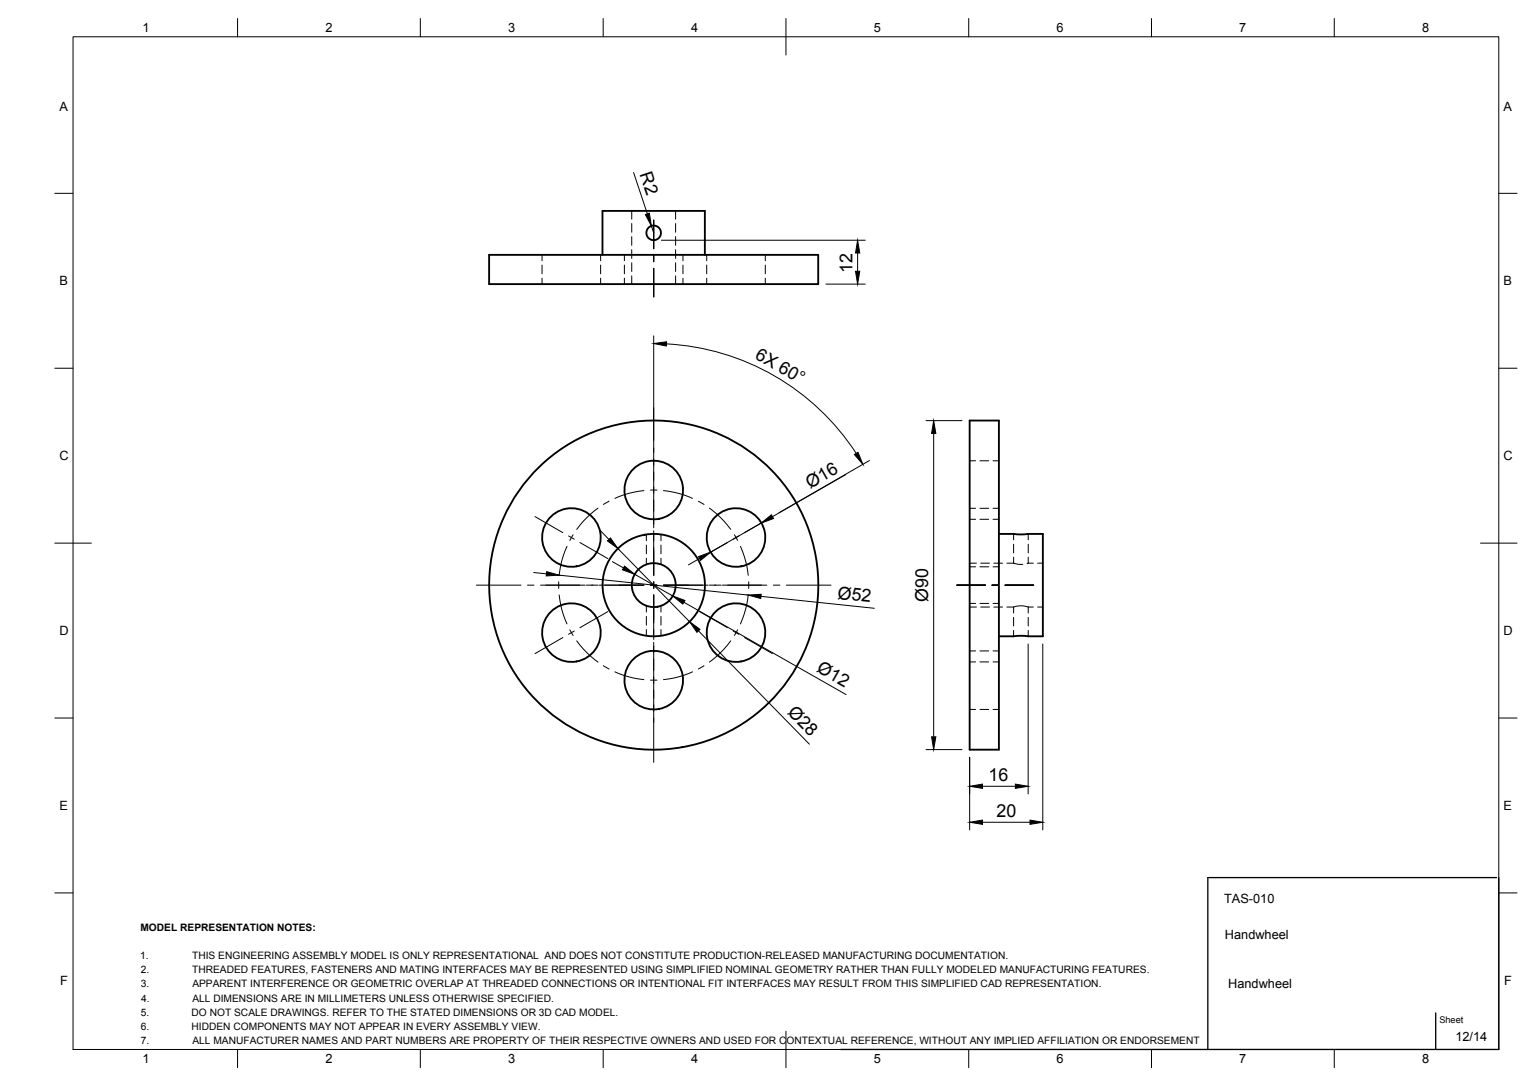
ISO-10303-21;
HEADER;
/* Generated by software containing ST-Developer
 * from STEP Tools, Inc. (www.steptools.com) 
 */

FILE_DESCRIPTION(
/* description */ (
'Independent keyed-quill tailstock, native coupled50mm slider andM16x2
 feed screw, conical dead center, bronze sleeves/thrust washers, cross
-pinned handwheel and bolted guide key. Custom center taper; no standa
rd taper compatibility, machine-bed compatibility or load rating assig
ned.'),
/* implementation_level */ '2;1');

FILE_NAME(
/* name */ 'Handwheel.step',
/* time_stamp */ '2026-11-14T07:17:36-08:00',
/* author */ (''),
/* organization */ (''),
/* preprocessor_version */ 'ST-DEVELOPER v20.2',
/* originating_system */ 'Autodesk Translation Framework v15.17.0.0',
/* authorisation */ '');

FILE_SCHEMA (('AUTOMOTIVE_DESIGN { 1 0 10303 214 3 1 1 }'));
ENDSEC;

DATA;
#10=MECHANICAL_DESIGN_GEOMETRIC_PRESENTATION_REPRESENTATION('',(#162),#289387);
#128=SHAPE_REPRESENTATION_RELATIONSHIP('SRR','None',#289463,#145);
#145=ADVANCED_BREP_SHAPE_REPRESENTATION('',(#179),#289379);
#162=STYLED_ITEM('',(#289549),#179);
#179=MANIFOLD_SOLID_BREP('Body1',#16850);
#243=FACE_BOUND('',#1657,.T.);
#244=FACE_BOUND('',#1659,.T.);
#245=FACE_BOUND('',#1661,.T.);
#246=FACE_BOUND('',#1664,.T.);
#247=FACE_BOUND('',#1665,.T.);
#248=FACE_BOUND('',#1666,.T.);
#249=FACE_BOUND('',#1667,.T.);
#250=FACE_BOUND('',#1668,.T.);
#251=FACE_BOUND('',#1669,.T.);
#252=FACE_BOUND('',#1670,.T.);
#253=FACE_BOUND('',#1672,.T.);
#254=FACE_BOUND('',#1673,.T.);
#255=FACE_BOUND('',#1674,.T.);
#256=FACE_BOUND('',#1675,.T.);
#257=FACE_BOUND('',#1676,.T.);
#258=FACE_BOUND('',#1677,.T.);
#259=FACE_BOUND('',#1678,.T.);
#377=PLANE('',#17691);
#378=PLANE('',#17698);
#379=PLANE('',#17699);
#942=FACE_OUTER_BOUND('',#1648,.T.);
#943=FACE_OUTER_BOUND('',#1649,.T.);
#944=FACE_OUTER_BOUND('',#1650,.T.);
#945=FACE_OUTER_BOUND('',#1651,.T.);
#946=FACE_OUTER_BOUND('',#1652,.T.);
#947=FACE_OUTER_BOUND('',#1653,.T.);
#948=FACE_OUTER_BOUND('',#1654,.T.);
#949=FACE_OUTER_BOUND('',#1655,.T.);
#950=FACE_OUTER_BOUND('',#1656,.T.);
#951=FACE_OUTER_BOUND('',#1658,.T.);
#952=FACE_OUTER_BOUND('',#1660,.T.);
#953=FACE_OUTER_BOUND('',#1662,.T.);
#954=FACE_OUTER_BOUND('',#1663,.T.);
#955=FACE_OUTER_BOUND('',#1671,.T.);
#1648=EDGE_LOOP('',(#14691,#14692,#14693,#14694,#14695,#14696));
#1649=EDGE_LOOP('',(#14697,#14698,#14699,#14700,#14701,#14702,#14703,#14704));
#1650=EDGE_LOOP('',(#14705,#14706,#14707,#14708));
#1651=EDGE_LOOP('',(#14709,#14710,#14711,#14712));
#1652=EDGE_LOOP('',(#14713,#14714,#14715,#14716));
#1653=EDGE_LOOP('',(#14717,#14718,#14719,#14720));
#1654=EDGE_LOOP('',(#14721,#14722,#14723,#14724));
#1655=EDGE_LOOP('',(#14725,#14726,#14727,#14728));
#1656=EDGE_LOOP('',(#14729,#14730,#14731,#14732,#14733,#14734,#14735,#14736,
#14737));
#1657=EDGE_LOOP('',(#14738,#14739,#14740));
#1658=EDGE_LOOP('',(#14741));
#1659=EDGE_LOOP('',(#14742));
#1660=EDGE_LOOP('',(#14743,#14744,#14745,#14746,#14747,#14748,#14749,#14750,
#14751));
#1661=EDGE_LOOP('',(#14752));
#1662=EDGE_LOOP('',(#14753,#14754,#14755,#14756));
#1663=EDGE_LOOP('',(#14757));
#1664=EDGE_LOOP('',(#14758));
#1665=EDGE_LOOP('',(#14759));
#1666=EDGE_LOOP('',(#14760));
#1667=EDGE_LOOP('',(#14761));
#1668=EDGE_LOOP('',(#14762));
#1669=EDGE_LOOP('',(#14763));
#1670=EDGE_LOOP('',(#14764));
#1671=EDGE_LOOP('',(#14765));
#1672=EDGE_LOOP('',(#14766));
#1673=EDGE_LOOP('',(#14767));
#1674=EDGE_LOOP('',(#14768));
#1675=EDGE_LOOP('',(#14769));
#1676=EDGE_LOOP('',(#14770));
#1677=EDGE_LOOP('',(#14771));
#1678=EDGE_LOOP('',(#14772));
#1925=CIRCLE('',#17671,8.);
#1926=CIRCLE('',#17672,8.);
#1927=CIRCLE('',#17674,8.);
#1928=CIRCLE('',#17675,8.);
#1929=CIRCLE('',#17677,8.);
#1930=CIRCLE('',#17678,8.);
#1931=CIRCLE('',#17680,8.);
#1932=CIRCLE('',#17681,8.);
#1933=CIRCLE('',#17683,8.);
#1934=CIRCLE('',#17684,8.);
#1935=CIRCLE('',#17686,8.);
#1936=CIRCLE('',#17687,8.);
#1937=CIRCLE('',#17689,14.);
#1938=CIRCLE('',#17690,14.);
#1939=CIRCLE('',#17692,6.);
#1940=CIRCLE('',#17694,6.);
#1941=CIRCLE('',#17696,45.);
#1942=CIRCLE('',#17697,45.);
#3636=B_SPLINE_CURVE_WITH_KNOTS('',3,(#247043,#247044,#247045,#247046,#247047,
#247048,#247049,#247050,#247051,#247052),.UNSPECIFIED.,.F.,.F.,(4,2,2,2,
4),(0.905379612473188,0.980827373439309,1.05627513440543,1.13172397551817,
1.20717281663092),.UNSPECIFIED.);
#3637=B_SPLINE_CURVE_WITH_KNOTS('',3,(#247054,#247055,#247056,#247057,#247058,
#247059,#247060,#247061,#247062,#247063,#247064,#247065,#247066,#247067,
#247068,#247069,#247070,#247071),.UNSPECIFIED.,.F.,.F.,(4,2,2,2,2,2,2,2,
4),(0.301793204157729,0.377240965123851,0.452688726089972,0.528137567202715,
0.603586408315459,0.679035249428202,0.754484090540945,0.829931851507066,
0.905379612473188),.UNSPECIFIED.);
#3638=B_SPLINE_CURVE_WITH_KNOTS('',3,(#247072,#247073,#247074,#247075,#247076,
#247077,#247078,#247079,#247080,#247081),.UNSPECIFIED.,.F.,.F.,(4,2,2,2,
4),(1.20717281663092,1.28262165774366,1.3580704988564,1.43351825982252,
1.50896602078865),.UNSPECIFIED.);
#3639=B_SPLINE_CURVE_WITH_KNOTS('',3,(#247084,#247085,#247086,#247087,#247088,
#247089,#247090,#247091,#247092,#247093,#247094,#247095,#247096,#247097,
#247098,#247099,#247100,#247101,#247102,#247103,#247104,#247105,#247106,
#247107,#247108,#247109,#247110,#247111,#247112,#247113,#247114,#247115,
#247116,#247117),.UNSPECIFIED.,.T.,.F.,(4,2,2,2,2,2,2,2,2,2,2,2,2,2,2,2,
4),(-1.21552023492118,-1.13953259867645,-1.06354496243171,-0.987592569311299,
-0.911640176190888,-0.835687783070478,-0.759735389950067,-0.683747753705329,
-0.607760117460592,-0.531772481215855,-0.455784844971118,-0.379832451850707,
-0.303880058730296,-0.227927665609885,-0.151975272489474,-0.0759876362447371,
0.),.UNSPECIFIED.);
#3640=B_SPLINE_CURVE_WITH_KNOTS('',3,(#247121,#247122,#247123,#247124,#247125,
#247126,#247127,#247128,#247129,#247130),.UNSPECIFIED.,.F.,.F.,(4,2,2,2,
4),(-0.303880058730296,-0.227927665609886,-0.151975272489475,-0.0759876362447375,
0.),.UNSPECIFIED.);
#3641=B_SPLINE_CURVE_WITH_KNOTS('',3,(#247132,#247133,#247134,#247135,#247136,
#247137,#247138,#247139,#247140,#247141,#247142,#247143,#247144,#247145,
#247146,#247147,#247148,#247149),.UNSPECIFIED.,.F.,.F.,(4,2,2,2,2,2,2,2,
4),(-0.911640176190889,-0.835687783070478,-0.759735389950067,-0.68374775370533,
-0.607760117460593,-0.531772481215855,-0.455784844971118,-0.379832451850707,
-0.303880058730296),.UNSPECIFIED.);
#3642=B_SPLINE_CURVE_WITH_KNOTS('',3,(#247150,#247151,#247152,#247153,#247154,
#247155,#247156,#247157,#247158,#247159),.UNSPECIFIED.,.F.,.F.,(4,2,2,2,
4),(0.,0.0759876362447371,0.151975272489474,0.227927665609885,0.303880058730296),
 .UNSPECIFIED.);
#3643=B_SPLINE_CURVE_WITH_KNOTS('',3,(#247163,#247164,#247165,#247166,#247167,
#247168,#247169,#247170,#247171,#247172),.UNSPECIFIED.,.F.,.F.,(4,2,2,2,
4),(0.905379612473188,0.980827373439309,1.05627513440543,1.13172397551817,
1.20717281663092),.UNSPECIFIED.);
#3644=B_SPLINE_CURVE_WITH_KNOTS('',3,(#247174,#247175,#247176,#247177,#247178,
#247179,#247180,#247181,#247182,#247183,#247184,#247185,#247186,#247187,
#247188,#247189,#247190,#247191),.UNSPECIFIED.,.F.,.F.,(4,2,2,2,2,2,2,2,
4),(0.301793204157729,0.377240965123851,0.452688726089972,0.528137567202715,
0.603586408315459,0.679035249428202,0.754484090540945,0.829931851507066,
0.905379612473188),.UNSPECIFIED.);
#3645=B_SPLINE_CURVE_WITH_KNOTS('',3,(#247192,#247193,#247194,#247195,#247196,
#247197,#247198,#247199,#247200,#247201),.UNSPECIFIED.,.F.,.F.,(4,2,2,2,
4),(1.20717281663092,1.28262165774366,1.3580704988564,1.43351825982252,
1.50896602078865),.UNSPECIFIED.);
#4443=LINE('',#247083,#5080);
#4444=LINE('',#247161,#5081);
#4445=LINE('',#247206,#5082);
#4446=LINE('',#247212,#5083);
#4447=LINE('',#247218,#5084);
#4448=LINE('',#247224,#5085);
#4449=LINE('',#247230,#5086);
#4450=LINE('',#247236,#5087);
#4451=LINE('',#247241,#5088);
#4452=LINE('',#247243,#5089);
#4453=LINE('',#247251,#5090);
#4454=LINE('',#247252,#5091);
#4455=LINE('',#247257,#5092);
#5080=VECTOR('',#19637,2.);
#5081=VECTOR('',#19640,2.);
#5082=VECTOR('',#19645,8.);
#5083=VECTOR('',#19652,8.);
#5084=VECTOR('',#19659,8.);
#5085=VECTOR('',#19666,8.);
#5086=VECTOR('',#19673,8.);
#5087=VECTOR('',#19680,8.);
#5088=VECTOR('',#19687,14.);
#5089=VECTOR('',#19688,14.);
#5090=VECTOR('',#19699,6.);
#5091=VECTOR('',#19700,6.);
#5092=VECTOR('',#19705,45.);
#6995=VERTEX_POINT('',#247041);
#6996=VERTEX_POINT('',#247042);
#6997=VERTEX_POINT('',#247053);
#6998=VERTEX_POINT('',#247082);
#6999=VERTEX_POINT('',#247119);
#7000=VERTEX_POINT('',#247120);
#7001=VERTEX_POINT('',#247131);
#7002=VERTEX_POINT('',#247160);
#7003=VERTEX_POINT('',#247162);
#7004=VERTEX_POINT('',#247173);
#7005=VERTEX_POINT('',#247203);
#7006=VERTEX_POINT('',#247205);
#7007=VERTEX_POINT('',#247209);
#7008=VERTEX_POINT('',#247211);
#7009=VERTEX_POINT('',#247215);
#7010=VERTEX_POINT('',#247217);
#7011=VERTEX_POINT('',#247221);
#7012=VERTEX_POINT('',#247223);
#7013=VERTEX_POINT('',#247227);
#7014=VERTEX_POINT('',#247229);
#7015=VERTEX_POINT('',#247233);
#7016=VERTEX_POINT('',#247235);
#7017=VERTEX_POINT('',#247239);
#7018=VERTEX_POINT('',#247242);
#7019=VERTEX_POINT('',#247246);
#7020=VERTEX_POINT('',#247249);
#7021=VERTEX_POINT('',#247254);
#7022=VERTEX_POINT('',#247256);
#9657=EDGE_CURVE('',#6995,#6996,#3636,.T.);
#9658=EDGE_CURVE('',#6997,#6995,#3637,.T.);
#9659=EDGE_CURVE('',#6996,#6997,#3638,.T.);
#9660=EDGE_CURVE('',#6996,#6998,#4443,.T.);
#9661=EDGE_CURVE('',#6998,#6998,#3639,.T.);
#9662=EDGE_CURVE('',#6999,#7000,#3640,.T.);
#9663=EDGE_CURVE('',#7001,#6999,#3641,.T.);
#9664=EDGE_CURVE('',#7000,#7001,#3642,.T.);
#9665=EDGE_CURVE('',#7000,#7002,#4444,.T.);
#9666=EDGE_CURVE('',#7003,#7002,#3643,.T.);
#9667=EDGE_CURVE('',#7004,#7003,#3644,.T.);
#9668=EDGE_CURVE('',#7002,#7004,#3645,.T.);
#9669=EDGE_CURVE('',#7005,#7005,#1925,.T.);
#9670=EDGE_CURVE('',#7005,#7006,#4445,.T.);
#9671=EDGE_CURVE('',#7006,#7006,#1926,.T.);
#9672=EDGE_CURVE('',#7007,#7007,#1927,.T.);
#9673=EDGE_CURVE('',#7007,#7008,#4446,.T.);
#9674=EDGE_CURVE('',#7008,#7008,#1928,.T.);
#9675=EDGE_CURVE('',#7009,#7009,#1929,.T.);
#9676=EDGE_CURVE('',#7009,#7010,#4447,.T.);
#9677=EDGE_CURVE('',#7010,#7010,#1930,.T.);
#9678=EDGE_CURVE('',#7011,#7011,#1931,.T.);
#9679=EDGE_CURVE('',#7011,#7012,#4448,.T.);
#9680=EDGE_CURVE('',#7012,#7012,#1932,.T.);
#9681=EDGE_CURVE('',#7013,#7013,#1933,.T.);
#9682=EDGE_CURVE('',#7013,#7014,#4449,.T.);
#9683=EDGE_CURVE('',#7014,#7014,#1934,.T.);
#9684=EDGE_CURVE('',#7015,#7015,#1935,.T.);
#9685=EDGE_CURVE('',#7015,#7016,#4450,.T.);
#9686=EDGE_CURVE('',#7016,#7016,#1936,.T.);
#9687=EDGE_CURVE('',#7017,#7017,#1937,.T.);
#9688=EDGE_CURVE('',#7017,#7003,#4451,.T.);
#9689=EDGE_CURVE('',#7004,#7018,#4452,.T.);
#9690=EDGE_CURVE('',#7018,#7018,#1938,.T.);
#9691=EDGE_CURVE('',#7019,#7019,#1939,.T.);
#9692=EDGE_CURVE('',#7020,#7020,#1940,.T.);
#9693=EDGE_CURVE('',#7020,#6999,#4453,.T.);
#9694=EDGE_CURVE('',#7001,#7019,#4454,.T.);
#9695=EDGE_CURVE('',#7021,#7021,#1941,.F.);
#9696=EDGE_CURVE('',#7021,#7022,#4455,.T.);
#9697=EDGE_CURVE('',#7022,#7022,#1942,.F.);
#14691=ORIENTED_EDGE('',*,*,#9657,.F.);
#14692=ORIENTED_EDGE('',*,*,#9658,.F.);
#14693=ORIENTED_EDGE('',*,*,#9659,.F.);
#14694=ORIENTED_EDGE('',*,*,#9660,.T.);
#14695=ORIENTED_EDGE('',*,*,#9661,.F.);
#14696=ORIENTED_EDGE('',*,*,#9660,.F.);
#14697=ORIENTED_EDGE('',*,*,#9662,.F.);
#14698=ORIENTED_EDGE('',*,*,#9663,.F.);
#14699=ORIENTED_EDGE('',*,*,#9664,.F.);
#14700=ORIENTED_EDGE('',*,*,#9665,.T.);
#14701=ORIENTED_EDGE('',*,*,#9666,.F.);
#14702=ORIENTED_EDGE('',*,*,#9667,.F.);
#14703=ORIENTED_EDGE('',*,*,#9668,.F.);
#14704=ORIENTED_EDGE('',*,*,#9665,.F.);
#14705=ORIENTED_EDGE('',*,*,#9669,.F.);
#14706=ORIENTED_EDGE('',*,*,#9670,.T.);
#14707=ORIENTED_EDGE('',*,*,#9671,.F.);
#14708=ORIENTED_EDGE('',*,*,#9670,.F.);
#14709=ORIENTED_EDGE('',*,*,#9672,.F.);
#14710=ORIENTED_EDGE('',*,*,#9673,.T.);
#14711=ORIENTED_EDGE('',*,*,#9674,.F.);
#14712=ORIENTED_EDGE('',*,*,#9673,.F.);
#14713=ORIENTED_EDGE('',*,*,#9675,.F.);
#14714=ORIENTED_EDGE('',*,*,#9676,.T.);
#14715=ORIENTED_EDGE('',*,*,#9677,.F.);
#14716=ORIENTED_EDGE('',*,*,#9676,.F.);
#14717=ORIENTED_EDGE('',*,*,#9678,.F.);
#14718=ORIENTED_EDGE('',*,*,#9679,.T.);
#14719=ORIENTED_EDGE('',*,*,#9680,.F.);
#14720=ORIENTED_EDGE('',*,*,#9679,.F.);
#14721=ORIENTED_EDGE('',*,*,#9681,.F.);
#14722=ORIENTED_EDGE('',*,*,#9682,.T.);
#14723=ORIENTED_EDGE('',*,*,#9683,.F.);
#14724=ORIENTED_EDGE('',*,*,#9682,.F.);
#14725=ORIENTED_EDGE('',*,*,#9684,.F.);
#14726=ORIENTED_EDGE('',*,*,#9685,.T.);
#14727=ORIENTED_EDGE('',*,*,#9686,.F.);
#14728=ORIENTED_EDGE('',*,*,#9685,.F.);
#14729=ORIENTED_EDGE('',*,*,#9687,.F.);
#14730=ORIENTED_EDGE('',*,*,#9688,.T.);
#14731=ORIENTED_EDGE('',*,*,#9666,.T.);
#14732=ORIENTED_EDGE('',*,*,#9668,.T.);
#14733=ORIENTED_EDGE('',*,*,#9689,.T.);
#14734=ORIENTED_EDGE('',*,*,#9690,.F.);
#14735=ORIENTED_EDGE('',*,*,#9689,.F.);
#14736=ORIENTED_EDGE('',*,*,#9667,.T.);
#14737=ORIENTED_EDGE('',*,*,#9688,.F.);
#14738=ORIENTED_EDGE('',*,*,#9658,.T.);
#14739=ORIENTED_EDGE('',*,*,#9657,.T.);
#14740=ORIENTED_EDGE('',*,*,#9659,.T.);
#14741=ORIENTED_EDGE('',*,*,#9687,.T.);
#14742=ORIENTED_EDGE('',*,*,#9691,.T.);
#14743=ORIENTED_EDGE('',*,*,#9692,.T.);
#14744=ORIENTED_EDGE('',*,*,#9693,.T.);
#14745=ORIENTED_EDGE('',*,*,#9662,.T.);
#14746=ORIENTED_EDGE('',*,*,#9664,.T.);
#14747=ORIENTED_EDGE('',*,*,#9694,.T.);
#14748=ORIENTED_EDGE('',*,*,#9691,.F.);
#14749=ORIENTED_EDGE('',*,*,#9694,.F.);
#14750=ORIENTED_EDGE('',*,*,#9663,.T.);
#14751=ORIENTED_EDGE('',*,*,#9693,.F.);
#14752=ORIENTED_EDGE('',*,*,#9661,.T.);
#14753=ORIENTED_EDGE('',*,*,#9695,.F.);
#14754=ORIENTED_EDGE('',*,*,#9696,.T.);
#14755=ORIENTED_EDGE('',*,*,#9697,.T.);
#14756=ORIENTED_EDGE('',*,*,#9696,.F.);
#14757=ORIENTED_EDGE('',*,*,#9695,.T.);
#14758=ORIENTED_EDGE('',*,*,#9690,.T.);
#14759=ORIENTED_EDGE('',*,*,#9684,.T.);
#14760=ORIENTED_EDGE('',*,*,#9681,.T.);
#14761=ORIENTED_EDGE('',*,*,#9678,.T.);
#14762=ORIENTED_EDGE('',*,*,#9675,.T.);
#14763=ORIENTED_EDGE('',*,*,#9672,.T.);
#14764=ORIENTED_EDGE('',*,*,#9669,.T.);
#14765=ORIENTED_EDGE('',*,*,#9697,.F.);
#14766=ORIENTED_EDGE('',*,*,#9692,.F.);
#14767=ORIENTED_EDGE('',*,*,#9686,.T.);
#14768=ORIENTED_EDGE('',*,*,#9683,.T.);
#14769=ORIENTED_EDGE('',*,*,#9680,.T.);
#14770=ORIENTED_EDGE('',*,*,#9677,.T.);
#14771=ORIENTED_EDGE('',*,*,#9674,.T.);
#14772=ORIENTED_EDGE('',*,*,#9671,.T.);
#16117=CYLINDRICAL_SURFACE('',#17668,2.);
#16118=CYLINDRICAL_SURFACE('',#17669,2.);
#16119=CYLINDRICAL_SURFACE('',#17670,8.);
#16120=CYLINDRICAL_SURFACE('',#17673,8.);
#16121=CYLINDRICAL_SURFACE('',#17676,8.);
#16122=CYLINDRICAL_SURFACE('',#17679,8.);
#16123=CYLINDRICAL_SURFACE('',#17682,8.);
#16124=CYLINDRICAL_SURFACE('',#17685,8.);
#16125=CYLINDRICAL_SURFACE('',#17688,14.);
#16126=CYLINDRICAL_SURFACE('',#17693,6.);
#16127=CYLINDRICAL_SURFACE('',#17695,45.);
#16710=ADVANCED_FACE('',(#942),#16117,.F.);
#16711=ADVANCED_FACE('',(#943),#16118,.F.);
#16712=ADVANCED_FACE('',(#944),#16119,.F.);
#16713=ADVANCED_FACE('',(#945),#16120,.F.);
#16714=ADVANCED_FACE('',(#946),#16121,.F.);
#16715=ADVANCED_FACE('',(#947),#16122,.F.);
#16716=ADVANCED_FACE('',(#948),#16123,.F.);
#16717=ADVANCED_FACE('',(#949),#16124,.F.);
#16718=ADVANCED_FACE('',(#950,#243),#16125,.T.);
#16719=ADVANCED_FACE('',(#951,#244),#377,.T.);
#16720=ADVANCED_FACE('',(#952,#245),#16126,.F.);
#16721=ADVANCED_FACE('',(#953),#16127,.T.);
#16722=ADVANCED_FACE('',(#954,#246,#247,#248,#249,#250,#251,#252),#378,
 .T.);
#16723=ADVANCED_FACE('',(#955,#253,#254,#255,#256,#257,#258,#259),#379,
 .F.);
#16850=CLOSED_SHELL('',(#16710,#16711,#16712,#16713,#16714,#16715,#16716,
#16717,#16718,#16719,#16720,#16721,#16722,#16723));
#17667=AXIS2_PLACEMENT_3D('',#247039,#19633,#19634);
#17668=AXIS2_PLACEMENT_3D('',#247040,#19635,#19636);
#17669=AXIS2_PLACEMENT_3D('',#247118,#19638,#19639);
#17670=AXIS2_PLACEMENT_3D('',#247202,#19641,#19642);
#17671=AXIS2_PLACEMENT_3D('',#247204,#19643,#19644);
#17672=AXIS2_PLACEMENT_3D('',#247207,#19646,#19647);
#17673=AXIS2_PLACEMENT_3D('',#247208,#19648,#19649);
#17674=AXIS2_PLACEMENT_3D('',#247210,#19650,#19651);
#17675=AXIS2_PLACEMENT_3D('',#247213,#19653,#19654);
#17676=AXIS2_PLACEMENT_3D('',#247214,#19655,#19656);
#17677=AXIS2_PLACEMENT_3D('',#247216,#19657,#19658);
#17678=AXIS2_PLACEMENT_3D('',#247219,#19660,#19661);
#17679=AXIS2_PLACEMENT_3D('',#247220,#19662,#19663);
#17680=AXIS2_PLACEMENT_3D('',#247222,#19664,#19665);
#17681=AXIS2_PLACEMENT_3D('',#247225,#19667,#19668);
#17682=AXIS2_PLACEMENT_3D('',#247226,#19669,#19670);
#17683=AXIS2_PLACEMENT_3D('',#247228,#19671,#19672);
#17684=AXIS2_PLACEMENT_3D('',#247231,#19674,#19675);
#17685=AXIS2_PLACEMENT_3D('',#247232,#19676,#19677);
#17686=AXIS2_PLACEMENT_3D('',#247234,#19678,#19679);
#17687=AXIS2_PLACEMENT_3D('',#247237,#19681,#19682);
#17688=AXIS2_PLACEMENT_3D('',#247238,#19683,#19684);
#17689=AXIS2_PLACEMENT_3D('',#247240,#19685,#19686);
#17690=AXIS2_PLACEMENT_3D('',#247244,#19689,#19690);
#17691=AXIS2_PLACEMENT_3D('',#247245,#19691,#19692);
#17692=AXIS2_PLACEMENT_3D('',#247247,#19693,#19694);
#17693=AXIS2_PLACEMENT_3D('',#247248,#19695,#19696);
#17694=AXIS2_PLACEMENT_3D('',#247250,#19697,#19698);
#17695=AXIS2_PLACEMENT_3D('',#247253,#19701,#19702);
#17696=AXIS2_PLACEMENT_3D('',#247255,#19703,#19704);
#17697=AXIS2_PLACEMENT_3D('',#247258,#19706,#19707);
#17698=AXIS2_PLACEMENT_3D('',#247259,#19708,#19709);
#17699=AXIS2_PLACEMENT_3D('',#247260,#19710,#19711);
#19633=DIRECTION('axis',(0.,0.,1.));
#19634=DIRECTION('refdir',(1.,0.,0.));
#19635=DIRECTION('center_axis',(-1.,0.,0.));
#19636=DIRECTION('ref_axis',(0.,1.,0.));
#19637=DIRECTION('',(-1.,0.,0.));
#19638=DIRECTION('center_axis',(-1.,0.,0.));
#19639=DIRECTION('ref_axis',(0.,1.,0.));
#19640=DIRECTION('',(-1.,0.,0.));
#19641=DIRECTION('center_axis',(0.,0.,-1.));
#19642=DIRECTION('ref_axis',(1.,0.,0.));
#19643=DIRECTION('center_axis',(0.,0.,-1.));
#19644=DIRECTION('ref_axis',(1.,0.,0.));
#19645=DIRECTION('',(0.,0.,-1.));
#19646=DIRECTION('center_axis',(0.,0.,1.));
#19647=DIRECTION('ref_axis',(1.,0.,0.));
#19648=DIRECTION('center_axis',(0.,0.,-1.));
#19649=DIRECTION('ref_axis',(1.,0.,0.));
#19650=DIRECTION('center_axis',(0.,0.,-1.));
#19651=DIRECTION('ref_axis',(1.,0.,0.));
#19652=DIRECTION('',(0.,0.,-1.));
#19653=DIRECTION('center_axis',(0.,0.,1.));
#19654=DIRECTION('ref_axis',(1.,0.,0.));
#19655=DIRECTION('center_axis',(0.,0.,-1.));
#19656=DIRECTION('ref_axis',(1.,0.,0.));
#19657=DIRECTION('center_axis',(0.,0.,-1.));
#19658=DIRECTION('ref_axis',(1.,0.,0.));
#19659=DIRECTION('',(0.,0.,-1.));
#19660=DIRECTION('center_axis',(0.,0.,1.));
#19661=DIRECTION('ref_axis',(1.,0.,0.));
#19662=DIRECTION('center_axis',(0.,0.,-1.));
#19663=DIRECTION('ref_axis',(1.,0.,0.));
#19664=DIRECTION('center_axis',(0.,0.,-1.));
#19665=DIRECTION('ref_axis',(1.,0.,0.));
#19666=DIRECTION('',(0.,0.,-1.));
#19667=DIRECTION('center_axis',(0.,0.,1.));
#19668=DIRECTION('ref_axis',(1.,0.,0.));
#19669=DIRECTION('center_axis',(0.,0.,-1.));
#19670=DIRECTION('ref_axis',(1.,0.,0.));
#19671=DIRECTION('center_axis',(0.,0.,-1.));
#19672=DIRECTION('ref_axis',(1.,0.,0.));
#19673=DIRECTION('',(0.,0.,-1.));
#19674=DIRECTION('center_axis',(0.,0.,1.));
#19675=DIRECTION('ref_axis',(1.,0.,0.));
#19676=DIRECTION('center_axis',(0.,0.,-1.));
#19677=DIRECTION('ref_axis',(1.,0.,0.));
#19678=DIRECTION('center_axis',(0.,0.,-1.));
#19679=DIRECTION('ref_axis',(1.,0.,0.));
#19680=DIRECTION('',(0.,0.,-1.));
#19681=DIRECTION('center_axis',(0.,0.,1.));
#19682=DIRECTION('ref_axis',(1.,0.,0.));
#19683=DIRECTION('center_axis',(0.,0.,1.));
#19684=DIRECTION('ref_axis',(1.,0.,0.));
#19685=DIRECTION('center_axis',(0.,0.,1.));
#19686=DIRECTION('ref_axis',(1.,0.,0.));
#19687=DIRECTION('',(0.,0.,-1.));
#19688=DIRECTION('',(0.,0.,-1.));
#19689=DIRECTION('center_axis',(0.,0.,-1.));
#19690=DIRECTION('ref_axis',(1.,0.,0.));
#19691=DIRECTION('center_axis',(0.,0.,1.));
#19692=DIRECTION('ref_axis',(1.,0.,0.));
#19693=DIRECTION('center_axis',(0.,0.,-1.));
#19694=DIRECTION('ref_axis',(1.,0.,0.));
#19695=DIRECTION('center_axis',(0.,0.,1.));
#19696=DIRECTION('ref_axis',(1.,0.,0.));
#19697=DIRECTION('center_axis',(0.,0.,-1.));
#19698=DIRECTION('ref_axis',(1.,0.,0.));
#19699=DIRECTION('',(0.,0.,1.));
#19700=DIRECTION('',(0.,0.,1.));
#19701=DIRECTION('center_axis',(0.,0.,1.));
#19702=DIRECTION('ref_axis',(1.,0.,0.));
#19703=DIRECTION('center_axis',(0.,0.,-1.));
#19704=DIRECTION('ref_axis',(1.,0.,0.));
#19705=DIRECTION('',(0.,0.,-1.));
#19706=DIRECTION('center_axis',(0.,0.,-1.));
#19707=DIRECTION('ref_axis',(1.,0.,0.));
#19708=DIRECTION('center_axis',(0.,0.,1.));
#19709=DIRECTION('ref_axis',(1.,0.,0.));
#19710=DIRECTION('center_axis',(0.,0.,1.));
#19711=DIRECTION('ref_axis',(1.,0.,0.));
#247039=CARTESIAN_POINT('',(0.,0.,0.));
#247040=CARTESIAN_POINT('Origin',(-2.22044604925031E-15,0.,14.));
#247041=CARTESIAN_POINT('',(14.,0.,12.));
#247042=CARTESIAN_POINT('',(13.856406460551,-2.,14.));
#247043=CARTESIAN_POINT('Ctrl Pts',(14.,6.24500451351651E-16,12.));
#247044=CARTESIAN_POINT('Ctrl Pts',(14.,-0.251492536553737,12.));
#247045=CARTESIAN_POINT('Ctrl Pts',(13.992532457489,-0.519514815600169,
12.0503312082537));
#247046=CARTESIAN_POINT('Ctrl Pts',(13.965542073511,-1.01217331161422,12.2545461305954));
#247047=CARTESIAN_POINT('Ctrl Pts',(13.9463980317977,-1.23683805013847,
12.4084109253923));
#247048=CARTESIAN_POINT('Ctrl Pts',(13.9103782647342,-1.59159161400131,
12.7631644892551));
#247049=CARTESIAN_POINT('Ctrl Pts',(13.891148239315,-1.74545441720186,12.9878281297258));
#247050=CARTESIAN_POINT('Ctrl Pts',(13.8639606805058,-1.94966788779478,
13.4804828838555));
#247051=CARTESIAN_POINT('Ctrl Pts',(13.856406460551,-2.,13.7485038629575));
#247052=CARTESIAN_POINT('Ctrl Pts',(13.856406460551,-2.,14.));
#247053=CARTESIAN_POINT('',(14.,0.,16.));
#247054=CARTESIAN_POINT('Ctrl Pts',(14.,-2.77555756156289E-16,16.));
#247055=CARTESIAN_POINT('Ctrl Pts',(14.,0.251492536553738,16.));
#247056=CARTESIAN_POINT('Ctrl Pts',(13.992532457489,0.51951481560017,15.9496687917463));
#247057=CARTESIAN_POINT('Ctrl Pts',(13.965542073511,1.01217331161422,15.7454538694046));
#247058=CARTESIAN_POINT('Ctrl Pts',(13.9463980317977,1.23683805013847,15.5915890746077));
#247059=CARTESIAN_POINT('Ctrl Pts',(13.9103782647342,1.59159161400131,15.2368355107449));
#247060=CARTESIAN_POINT('Ctrl Pts',(13.891148239315,1.74545441720186,15.0121718702742));
#247061=CARTESIAN_POINT('Ctrl Pts',(13.8639606805058,1.94966788779478,14.5195171161445));
#247062=CARTESIAN_POINT('Ctrl Pts',(13.856406460551,2.,14.2514961370425));
#247063=CARTESIAN_POINT('Ctrl Pts',(13.856406460551,2.,13.7485038629575));
#247064=CARTESIAN_POINT('Ctrl Pts',(13.8639606805058,1.94966788779478,13.4804828838555));
#247065=CARTESIAN_POINT('Ctrl Pts',(13.891148239315,1.74545441720186,12.9878281297258));
#247066=CARTESIAN_POINT('Ctrl Pts',(13.9103782647342,1.59159161400131,12.7631644892551));
#247067=CARTESIAN_POINT('Ctrl Pts',(13.9463980317977,1.23683805013847,12.4084109253923));
#247068=CARTESIAN_POINT('Ctrl Pts',(13.965542073511,1.01217331161422,12.2545461305954));
#247069=CARTESIAN_POINT('Ctrl Pts',(13.992532457489,0.519514815600173,12.0503312082537));
#247070=CARTESIAN_POINT('Ctrl Pts',(14.,0.251492536553739,12.));
#247071=CARTESIAN_POINT('Ctrl Pts',(14.,6.41847686111419E-16,12.));
#247072=CARTESIAN_POINT('Ctrl Pts',(13.856406460551,-2.,14.));
#247073=CARTESIAN_POINT('Ctrl Pts',(13.856406460551,-2.,14.2514961370425));
#247074=CARTESIAN_POINT('Ctrl Pts',(13.8639606805058,-1.94966788779478,
14.5195171161445));
#247075=CARTESIAN_POINT('Ctrl Pts',(13.891148239315,-1.74545441720186,15.0121718702742));
#247076=CARTESIAN_POINT('Ctrl Pts',(13.9103782647342,-1.59159161400131,
15.2368355107449));
#247077=CARTESIAN_POINT('Ctrl Pts',(13.9463980317977,-1.23683805013847,
15.5915890746077));
#247078=CARTESIAN_POINT('Ctrl Pts',(13.965542073511,-1.01217331161422,15.7454538694046));
#247079=CARTESIAN_POINT('Ctrl Pts',(13.992532457489,-0.519514815600171,
15.9496687917463));
#247080=CARTESIAN_POINT('Ctrl Pts',(14.,-0.251492536553739,16.));
#247081=CARTESIAN_POINT('Ctrl Pts',(14.,5.03069808033274E-16,16.));
#247082=CARTESIAN_POINT('',(5.65685424949238,-2.,14.));
#247083=CARTESIAN_POINT('',(-2.22044604925031E-15,-2.,14.));
#247084=CARTESIAN_POINT('Ctrl Pts',(5.65685424949238,-2.,14.));
#247085=CARTESIAN_POINT('Ctrl Pts',(5.65685424949238,-2.,13.7467078791842));
#247086=CARTESIAN_POINT('Ctrl Pts',(5.67565356574251,-1.94898067853762,
13.477996053073));
#247087=CARTESIAN_POINT('Ctrl Pts',(5.74186082552466,-1.7443058152527,12.9858936400846));
#247088=CARTESIAN_POINT('Ctrl Pts',(5.78813771212597,-1.59074095999941,
12.7623138352532));
#247089=CARTESIAN_POINT('Ctrl Pts',(5.87374622031365,-1.23776803829002,
12.4093409135438));
#247090=CARTESIAN_POINT('Ctrl Pts',(5.9188739106068,-1.01415562391481,12.2557130277668));
#247091=CARTESIAN_POINT('Ctrl Pts',(5.98240475886912,-0.521932274441715,
12.0509911583939));
#247092=CARTESIAN_POINT('Ctrl Pts',(6.,-0.253174643734702,12.));
#247093=CARTESIAN_POINT('Ctrl Pts',(6.,0.253174643734703,12.));
#247094=CARTESIAN_POINT('Ctrl Pts',(5.98240475886912,0.521932274441715,
12.0509911583939));
#247095=CARTESIAN_POINT('Ctrl Pts',(5.9188739106068,1.01415562391481,12.2557130277668));
#247096=CARTESIAN_POINT('Ctrl Pts',(5.87374622031365,1.23776803829002,12.4093409135438));
#247097=CARTESIAN_POINT('Ctrl Pts',(5.78813771212597,1.59074095999941,12.7623138352532));
#247098=CARTESIAN_POINT('Ctrl Pts',(5.74186082552466,1.7443058152527,12.9858936400846));
#247099=CARTESIAN_POINT('Ctrl Pts',(5.67565356574251,1.94898067853762,13.477996053073));
#247100=CARTESIAN_POINT('Ctrl Pts',(5.65685424949238,2.,13.7467078791842));
#247101=CARTESIAN_POINT('Ctrl Pts',(5.65685424949238,2.,14.2532921208158));
#247102=CARTESIAN_POINT('Ctrl Pts',(5.67565356574251,1.94898067853763,14.522003946927));
#247103=CARTESIAN_POINT('Ctrl Pts',(5.74186082552466,1.74430581525271,15.0141063599154));
#247104=CARTESIAN_POINT('Ctrl Pts',(5.78813771212597,1.59074095999941,15.2376861647468));
#247105=CARTESIAN_POINT('Ctrl Pts',(5.87374622031365,1.23776803829002,15.5906590864562));
#247106=CARTESIAN_POINT('Ctrl Pts',(5.9188739106068,1.01415562391481,15.7442869722332));
#247107=CARTESIAN_POINT('Ctrl Pts',(5.98240475886912,0.521932274441714,
15.9490088416061));
#247108=CARTESIAN_POINT('Ctrl Pts',(6.,0.253174643734703,16.));
#247109=CARTESIAN_POINT('Ctrl Pts',(6.,-0.253174643734703,16.));
#247110=CARTESIAN_POINT('Ctrl Pts',(5.98240475886912,-0.521932274441715,
15.9490088416061));
#247111=CARTESIAN_POINT('Ctrl Pts',(5.9188739106068,-1.01415562391481,15.7442869722332));
#247112=CARTESIAN_POINT('Ctrl Pts',(5.87374622031365,-1.23776803829002,
15.5906590864562));
#247113=CARTESIAN_POINT('Ctrl Pts',(5.78813771212597,-1.59074095999941,
15.2376861647468));
#247114=CARTESIAN_POINT('Ctrl Pts',(5.74186082552466,-1.74430581525271,
15.0141063599154));
#247115=CARTESIAN_POINT('Ctrl Pts',(5.67565356574251,-1.94898067853763,
14.522003946927));
#247116=CARTESIAN_POINT('Ctrl Pts',(5.65685424949238,-2.,14.2532921208158));
#247117=CARTESIAN_POINT('Ctrl Pts',(5.65685424949238,-2.,14.));
#247118=CARTESIAN_POINT('Origin',(-2.22044604925031E-15,0.,14.));
#247119=CARTESIAN_POINT('',(-6.,-5.40866387341887E-16,12.));
#247120=CARTESIAN_POINT('',(-5.65685424949238,-2.,14.));
#247121=CARTESIAN_POINT('Ctrl Pts',(-6.,6.24500451351651E-16,12.));
#247122=CARTESIAN_POINT('Ctrl Pts',(-6.,-0.253174643734702,12.));
#247123=CARTESIAN_POINT('Ctrl Pts',(-5.98240475886912,-0.521932274441713,
12.0509911583939));
#247124=CARTESIAN_POINT('Ctrl Pts',(-5.9188739106068,-1.01415562391481,
12.2557130277668));
#247125=CARTESIAN_POINT('Ctrl Pts',(-5.87374622031365,-1.23776803829002,
12.4093409135438));
#247126=CARTESIAN_POINT('Ctrl Pts',(-5.78813771212597,-1.59074095999941,
12.7623138352532));
#247127=CARTESIAN_POINT('Ctrl Pts',(-5.74186082552466,-1.7443058152527,
12.9858936400846));
#247128=CARTESIAN_POINT('Ctrl Pts',(-5.67565356574251,-1.94898067853762,
13.477996053073));
#247129=CARTESIAN_POINT('Ctrl Pts',(-5.65685424949238,-2.,13.7467078791842));
#247130=CARTESIAN_POINT('Ctrl Pts',(-5.65685424949238,-2.,14.));
#247131=CARTESIAN_POINT('',(-6.,8.3634064009764E-17,16.));
#247132=CARTESIAN_POINT('Ctrl Pts',(-6.,-3.98986399474666E-16,16.));
#247133=CARTESIAN_POINT('Ctrl Pts',(-6.,0.253174643734703,16.));
#247134=CARTESIAN_POINT('Ctrl Pts',(-5.98240475886912,0.521932274441714,
15.9490088416061));
#247135=CARTESIAN_POINT('Ctrl Pts',(-5.9188739106068,1.01415562391481,15.7442869722332));
#247136=CARTESIAN_POINT('Ctrl Pts',(-5.87374622031365,1.23776803829002,
15.5906590864562));
#247137=CARTESIAN_POINT('Ctrl Pts',(-5.78813771212597,1.59074095999941,
15.2376861647468));
#247138=CARTESIAN_POINT('Ctrl Pts',(-5.74186082552466,1.74430581525271,
15.0141063599154));
#247139=CARTESIAN_POINT('Ctrl Pts',(-5.67565356574251,1.94898067853763,
14.522003946927));
#247140=CARTESIAN_POINT('Ctrl Pts',(-5.65685424949238,2.,14.2532921208158));
#247141=CARTESIAN_POINT('Ctrl Pts',(-5.65685424949238,2.,13.7467078791842));
#247142=CARTESIAN_POINT('Ctrl Pts',(-5.67565356574251,1.94898067853762,
13.477996053073));
#247143=CARTESIAN_POINT('Ctrl Pts',(-5.74186082552466,1.7443058152527,12.9858936400846));
#247144=CARTESIAN_POINT('Ctrl Pts',(-5.78813771212597,1.59074095999941,
12.7623138352532));
#247145=CARTESIAN_POINT('Ctrl Pts',(-5.87374622031365,1.23776803829002,
12.4093409135438));
#247146=CARTESIAN_POINT('Ctrl Pts',(-5.9188739106068,1.01415562391481,12.2557130277668));
#247147=CARTESIAN_POINT('Ctrl Pts',(-5.98240475886912,0.521932274441715,
12.0509911583939));
#247148=CARTESIAN_POINT('Ctrl Pts',(-6.,0.253174643734703,12.));
#247149=CARTESIAN_POINT('Ctrl Pts',(-6.,6.41847686111419E-16,12.));
#247150=CARTESIAN_POINT('Ctrl Pts',(-5.65685424949238,-2.,14.));
#247151=CARTESIAN_POINT('Ctrl Pts',(-5.65685424949238,-2.,14.2532921208158));
#247152=CARTESIAN_POINT('Ctrl Pts',(-5.67565356574251,-1.94898067853763,
14.522003946927));
#247153=CARTESIAN_POINT('Ctrl Pts',(-5.74186082552466,-1.74430581525271,
15.0141063599154));
#247154=CARTESIAN_POINT('Ctrl Pts',(-5.78813771212597,-1.59074095999941,
15.2376861647468));
#247155=CARTESIAN_POINT('Ctrl Pts',(-5.87374622031365,-1.23776803829002,
15.5906590864562));
#247156=CARTESIAN_POINT('Ctrl Pts',(-5.9188739106068,-1.01415562391481,
15.7442869722332));
#247157=CARTESIAN_POINT('Ctrl Pts',(-5.98240475886912,-0.521932274441715,
15.9490088416061));
#247158=CARTESIAN_POINT('Ctrl Pts',(-6.,-0.253174643734703,16.));
#247159=CARTESIAN_POINT('Ctrl Pts',(-6.,-3.98986399474666E-16,16.));
#247160=CARTESIAN_POINT('',(-13.856406460551,-2.,14.));
#247161=CARTESIAN_POINT('',(-2.22044604925031E-15,-2.,14.));
#247162=CARTESIAN_POINT('',(-14.,0.,16.));
#247163=CARTESIAN_POINT('Ctrl Pts',(-14.,-3.46944695195361E-16,16.));
#247164=CARTESIAN_POINT('Ctrl Pts',(-14.,-0.251492536553739,16.));
#247165=CARTESIAN_POINT('Ctrl Pts',(-13.992532457489,-0.519514815600171,
15.9496687917463));
#247166=CARTESIAN_POINT('Ctrl Pts',(-13.965542073511,-1.01217331161422,
15.7454538694046));
#247167=CARTESIAN_POINT('Ctrl Pts',(-13.9463980317977,-1.23683805013847,
15.5915890746077));
#247168=CARTESIAN_POINT('Ctrl Pts',(-13.9103782647342,-1.59159161400131,
15.2368355107449));
#247169=CARTESIAN_POINT('Ctrl Pts',(-13.891148239315,-1.74545441720187,
15.0121718702742));
#247170=CARTESIAN_POINT('Ctrl Pts',(-13.8639606805058,-1.94966788779478,
14.5195171161445));
#247171=CARTESIAN_POINT('Ctrl Pts',(-13.856406460551,-2.,14.2514961370425));
#247172=CARTESIAN_POINT('Ctrl Pts',(-13.856406460551,-2.,14.));
#247173=CARTESIAN_POINT('',(-14.,0.,12.));
#247174=CARTESIAN_POINT('Ctrl Pts',(-14.,6.07153216591882E-16,12.));
#247175=CARTESIAN_POINT('Ctrl Pts',(-14.,0.251492536553739,12.));
#247176=CARTESIAN_POINT('Ctrl Pts',(-13.992532457489,0.519514815600171,
12.0503312082537));
#247177=CARTESIAN_POINT('Ctrl Pts',(-13.965542073511,1.01217331161422,12.2545461305954));
#247178=CARTESIAN_POINT('Ctrl Pts',(-13.9463980317977,1.23683805013847,
12.4084109253923));
#247179=CARTESIAN_POINT('Ctrl Pts',(-13.9103782647342,1.59159161400131,
12.7631644892551));
#247180=CARTESIAN_POINT('Ctrl Pts',(-13.891148239315,1.74545441720186,12.9878281297258));
#247181=CARTESIAN_POINT('Ctrl Pts',(-13.8639606805058,1.94966788779478,
13.4804828838555));
#247182=CARTESIAN_POINT('Ctrl Pts',(-13.856406460551,2.,13.7485038629575));
#247183=CARTESIAN_POINT('Ctrl Pts',(-13.856406460551,2.,14.2514961370425));
#247184=CARTESIAN_POINT('Ctrl Pts',(-13.8639606805058,1.94966788779478,
14.5195171161445));
#247185=CARTESIAN_POINT('Ctrl Pts',(-13.891148239315,1.74545441720186,15.0121718702742));
#247186=CARTESIAN_POINT('Ctrl Pts',(-13.9103782647342,1.59159161400131,
15.2368355107449));
#247187=CARTESIAN_POINT('Ctrl Pts',(-13.9463980317977,1.23683805013847,
15.5915890746077));
#247188=CARTESIAN_POINT('Ctrl Pts',(-13.965542073511,1.01217331161422,15.7454538694046));
#247189=CARTESIAN_POINT('Ctrl Pts',(-13.992532457489,0.51951481560017,15.9496687917463));
#247190=CARTESIAN_POINT('Ctrl Pts',(-14.,0.251492536553738,16.));
#247191=CARTESIAN_POINT('Ctrl Pts',(-14.,-2.77555756156289E-16,16.));
#247192=CARTESIAN_POINT('Ctrl Pts',(-13.856406460551,-2.,14.));
#247193=CARTESIAN_POINT('Ctrl Pts',(-13.856406460551,-2.,13.7485038629575));
#247194=CARTESIAN_POINT('Ctrl Pts',(-13.8639606805058,-1.94966788779478,
13.4804828838555));
#247195=CARTESIAN_POINT('Ctrl Pts',(-13.891148239315,-1.74545441720186,
12.9878281297258));
#247196=CARTESIAN_POINT('Ctrl Pts',(-13.9103782647342,-1.59159161400131,
12.7631644892551));
#247197=CARTESIAN_POINT('Ctrl Pts',(-13.9463980317977,-1.23683805013847,
12.4084109253923));
#247198=CARTESIAN_POINT('Ctrl Pts',(-13.965542073511,-1.01217331161422,
12.2545461305954));
#247199=CARTESIAN_POINT('Ctrl Pts',(-13.992532457489,-0.519514815600169,
12.0503312082537));
#247200=CARTESIAN_POINT('Ctrl Pts',(-14.,-0.251492536553737,12.));
#247201=CARTESIAN_POINT('Ctrl Pts',(-14.,7.11236625150491E-16,12.));
#247202=CARTESIAN_POINT('Origin',(-13.,-22.5166604983954,4.));
#247203=CARTESIAN_POINT('',(-21.,-22.5166604983954,8.));
#247204=CARTESIAN_POINT('Origin',(-13.,-22.5166604983954,8.));
#247205=CARTESIAN_POINT('',(-21.,-22.5166604983954,0.));
#247206=CARTESIAN_POINT('',(-21.,-22.5166604983954,4.));
#247207=CARTESIAN_POINT('Origin',(-13.,-22.5166604983954,0.));
#247208=CARTESIAN_POINT('Origin',(-13.,22.5166604983954,4.));
#247209=CARTESIAN_POINT('',(-21.,22.5166604983954,8.));
#247210=CARTESIAN_POINT('Origin',(-13.,22.5166604983954,8.));
#247211=CARTESIAN_POINT('',(-21.,22.5166604983954,0.));
#247212=CARTESIAN_POINT('',(-21.,22.5166604983954,4.));
#247213=CARTESIAN_POINT('Origin',(-13.,22.5166604983954,0.));
#247214=CARTESIAN_POINT('Origin',(26.,0.,4.));
#247215=CARTESIAN_POINT('',(18.,9.79717439317883E-16,8.));
#247216=CARTESIAN_POINT('Origin',(26.,0.,8.));
#247217=CARTESIAN_POINT('',(18.,9.79717439317883E-16,0.));
#247218=CARTESIAN_POINT('',(18.,9.79717439317883E-16,4.));
#247219=CARTESIAN_POINT('Origin',(26.,0.,0.));
#247220=CARTESIAN_POINT('Origin',(13.,22.5166604983954,4.));
#247221=CARTESIAN_POINT('',(5.,22.5166604983954,8.));
#247222=CARTESIAN_POINT('Origin',(13.,22.5166604983954,8.));
#247223=CARTESIAN_POINT('',(5.,22.5166604983954,0.));
#247224=CARTESIAN_POINT('',(5.,22.5166604983954,4.));
#247225=CARTESIAN_POINT('Origin',(13.,22.5166604983954,0.));
#247226=CARTESIAN_POINT('Origin',(-26.,3.18408167778312E-15,4.));
#247227=CARTESIAN_POINT('',(-34.,4.163799117101E-15,8.));
#247228=CARTESIAN_POINT('Origin',(-26.,3.18408167778312E-15,8.));
#247229=CARTESIAN_POINT('',(-34.,4.163799117101E-15,0.));
#247230=CARTESIAN_POINT('',(-34.,4.163799117101E-15,4.));
#247231=CARTESIAN_POINT('Origin',(-26.,3.18408167778312E-15,0.));
#247232=CARTESIAN_POINT('Origin',(13.,-22.5166604983954,4.));
#247233=CARTESIAN_POINT('',(5.,-22.5166604983954,8.));
#247234=CARTESIAN_POINT('Origin',(13.,-22.5166604983954,8.));
#247235=CARTESIAN_POINT('',(5.,-22.5166604983954,0.));
#247236=CARTESIAN_POINT('',(5.,-22.5166604983954,4.));
#247237=CARTESIAN_POINT('Origin',(13.,-22.5166604983954,0.));
#247238=CARTESIAN_POINT('Origin',(0.,0.,0.));
#247239=CARTESIAN_POINT('',(-14.,-1.71450551880629E-15,20.));
#247240=CARTESIAN_POINT('Origin',(0.,0.,20.));
#247241=CARTESIAN_POINT('',(-14.,-1.71450551880629E-15,0.));
#247242=CARTESIAN_POINT('',(-14.,1.71450551880629E-15,8.));
#247243=CARTESIAN_POINT('',(-14.,-1.71450551880629E-15,0.));
#247244=CARTESIAN_POINT('Origin',(0.,0.,8.));
#247245=CARTESIAN_POINT('Origin',(0.,0.,20.));
#247246=CARTESIAN_POINT('',(-6.,-7.34788079488412E-16,20.));
#247247=CARTESIAN_POINT('Origin',(0.,0.,20.));
#247248=CARTESIAN_POINT('Origin',(0.,0.,0.));
#247249=CARTESIAN_POINT('',(-6.,-7.34788079488412E-16,0.));
#247250=CARTESIAN_POINT('Origin',(0.,0.,0.));
#247251=CARTESIAN_POINT('',(-6.,-7.34788079488412E-16,0.));
#247252=CARTESIAN_POINT('',(-6.,-7.34788079488412E-16,0.));
#247253=CARTESIAN_POINT('Origin',(0.,0.,0.));
#247254=CARTESIAN_POINT('',(-45.,5.51091059616309E-15,8.));
#247255=CARTESIAN_POINT('Origin',(0.,0.,8.));
#247256=CARTESIAN_POINT('',(-45.,5.51091059616309E-15,0.));
#247257=CARTESIAN_POINT('',(-45.,-5.51091059616309E-15,0.));
#247258=CARTESIAN_POINT('Origin',(0.,0.,0.));
#247259=CARTESIAN_POINT('Origin',(0.,0.,8.));
#247260=CARTESIAN_POINT('Origin',(0.,0.,0.));
#289360=UNCERTAINTY_MEASURE_WITH_UNIT(LENGTH_MEASURE(0.01),#289388,
'DISTANCE_ACCURACY_VALUE',
'Maximum model space distance between geometric entities at asserted c
onnectivities');
#289368=UNCERTAINTY_MEASURE_WITH_UNIT(LENGTH_MEASURE(0.01),#289388,
'DISTANCE_ACCURACY_VALUE',
'Maximum model space distance between geometric entities at asserted c
onnectivities');
#289379=(
GEOMETRIC_REPRESENTATION_CONTEXT(3)
GLOBAL_UNCERTAINTY_ASSIGNED_CONTEXT((#289360))
GLOBAL_UNIT_ASSIGNED_CONTEXT((#289388,#289390,#289391))
REPRESENTATION_CONTEXT('','3D')
);
#289387=(
GEOMETRIC_REPRESENTATION_CONTEXT(3)
GLOBAL_UNCERTAINTY_ASSIGNED_CONTEXT((#289368))
GLOBAL_UNIT_ASSIGNED_CONTEXT((#289388,#289390,#289391))
REPRESENTATION_CONTEXT('','3D')
);
#289388=(
LENGTH_UNIT()
NAMED_UNIT(*)
SI_UNIT(.MILLI.,.METRE.)
);
#289390=(
NAMED_UNIT(*)
PLANE_ANGLE_UNIT()
SI_UNIT($,.RADIAN.)
);
#289391=(
NAMED_UNIT(*)
SI_UNIT($,.STERADIAN.)
SOLID_ANGLE_UNIT()
);
#289402=SHAPE_DEFINITION_REPRESENTATION(#289420,#289463);
#289420=PRODUCT_DEFINITION_SHAPE('',$,#289482);
#289463=SHAPE_REPRESENTATION('',(#17667),#289379);
#289471=PRODUCT_DEFINITION_CONTEXT('part definition',#289527,'design');
#289482=PRODUCT_DEFINITION('Handwheel','Handwheel',#289500,#289471);
#289500=PRODUCT_DEFINITION_FORMATION('',$,#289539);
#289527=APPLICATION_CONTEXT(
'Core Data for Automotive Mechanical Design Process');
#289528=PRODUCT_CONTEXT('part definition',#289527,'mechanical');
#289539=PRODUCT('Handwheel','Handwheel','Handwheel',(#289528));
#289549=PRESENTATION_STYLE_ASSIGNMENT((#289556));
#289556=SURFACE_STYLE_USAGE(.BOTH.,#289563);
#289563=SURFACE_SIDE_STYLE('',(#289570));
#289570=SURFACE_STYLE_FILL_AREA(#289577);
#289577=FILL_AREA_STYLE('Opaque(23,69,131)',(#289584));
#289584=FILL_AREA_STYLE_COLOUR('Opaque(23,69,131)',#289591);
#289591=COLOUR_RGB('Opaque(23,69,131)',0.0901960784313725,0.270588235294118,
0.513725490196078);
ENDSEC;
END-ISO-10303-21;
